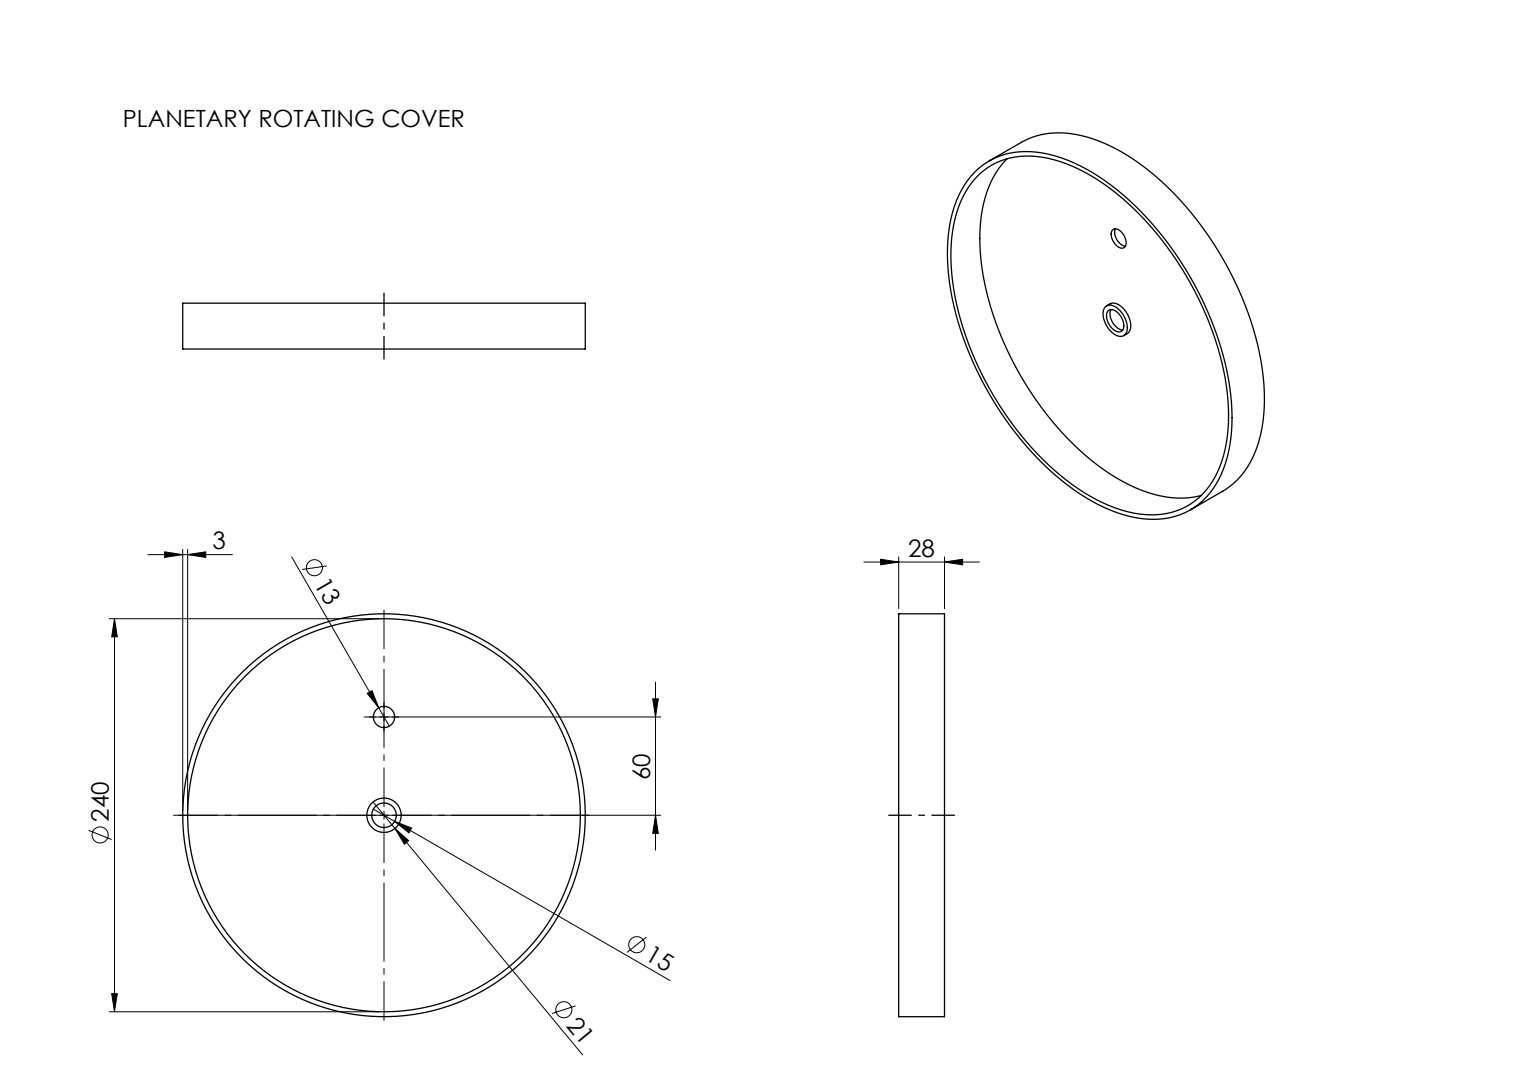
ISO-10303-21;
HEADER;
FILE_DESCRIPTION (('STEP AP214'),
    '1' );
FILE_NAME ('planetary rotating cover.step',
    '2026-09-30T13:58:28',
    ( '' ),
    ( '' ),
    'SwSTEP 2.0',
    'SolidWorks 2026',
    '' );
FILE_SCHEMA (( 'AUTOMOTIVE_DESIGN' ));
ENDSEC;

DATA;
#96=ORIENTED_EDGE ( 'NONE', *, *, #16353, .T. ) ;
#109=DIRECTION ( 'NONE',  ( -0.000000000000000000, -0.000000000000000000, 1.000000000000000000 ) ) ;
#161=ORIENTED_EDGE ( 'NONE', *, *, #12699, .T. ) ;
#178=ORIENTED_EDGE ( 'NONE', *, *, #6724, .F. ) ;
#209=EDGE_CURVE ( 'NONE', #16392, #6661, #15284, .T. ) ;
#268=CARTESIAN_POINT ( 'NONE',  ( 120.0000000000000000, 0.000000000000000000, -3.000000000000000000 ) ) ;
#330=CIRCLE ( 'NONE', #4199, 123.0000000000000000 ) ;
#469=CIRCLE ( 'NONE', #10677, 10.49999999999999822 ) ;
#487=CARTESIAN_POINT ( 'NONE',  ( 0.000000000000000000, 0.000000000000000000, 3.000000000000000000 ) ) ;
#587=FACE_OUTER_BOUND ( 'NONE', #12213, .T. ) ;
#707=DIRECTION ( 'NONE',  ( 0.000000000000000000, 0.000000000000000000, 1.000000000000000000 ) ) ;
#787=CARTESIAN_POINT ( 'NONE',  ( 0.000000000000000000, 0.000000000000000000, 25.00000000000000000 ) ) ;
#790=DIRECTION ( 'NONE',  ( -0.000000000000000000, -0.000000000000000000, -1.000000000000000000 ) ) ;
#853=ORIENTED_EDGE ( 'NONE', *, *, #4633, .T. ) ;
#891=FACE_OUTER_BOUND ( 'NONE', #4555, .T. ) ;
#949=FACE_OUTER_BOUND ( 'NONE', #6336, .T. ) ;
#1071=CARTESIAN_POINT ( 'NONE',  ( 6.499999999999984901, 60.00000000000001421, -3.000000000000000000 ) ) ;
#1097=EDGE_CURVE ( 'NONE', #6661, #9836, #21450, .T. ) ;
#1153=MECHANICAL_DESIGN_GEOMETRIC_PRESENTATION_REPRESENTATION('',(#14569),#20227);
#1202=DIRECTION ( 'NONE',  ( 0.000000000000000000, 0.000000000000000000, 1.000000000000000000 ) ) ;
#1264=CLOSED_SHELL ( 'NONE', ( #11800, #19951, #12732, #8634, #1598, #8913, #1358, #1778, #18719, #8874, #10287, #11609, #3169, #12589, #21642 ) ) ;
#1356=CYLINDRICAL_SURFACE ( 'NONE', #13917, 120.0000000000000000 ) ;
#1358=ADVANCED_FACE ( 'NONE', ( #13091 ), #3256, .T. ) ;
#1431=DIRECTION ( 'NONE',  ( 1.000000000000000000, 0.000000000000000000, 0.000000000000000000 ) ) ;
#1460=DIRECTION ( 'NONE',  ( 0.000000000000000000, 0.000000000000000000, 1.000000000000000000 ) ) ;
#1466=DIRECTION ( 'NONE',  ( 0.000000000000000000, 0.000000000000000000, 1.000000000000000000 ) ) ;
#1469=ORIENTED_EDGE ( 'NONE', *, *, #19172, .F. ) ;
#1491=EDGE_CURVE ( 'NONE', #2109, #20211, #15614, .T. ) ;
#1495=UNCERTAINTY_MEASURE_WITH_UNIT (LENGTH_MEASURE( 1.000000000000000082E-05 ), #15175, 'distance_accuracy_value', 'NONE');
#1560=AXIS2_PLACEMENT_3D ( 'NONE', #18307, #3156, #9890 ) ;
#1575=DIRECTION ( 'NONE',  ( -0.000000000000000000, -0.000000000000000000, 1.000000000000000000 ) ) ;
#1580=ORIENTED_EDGE ( 'NONE', *, *, #18346, .T. ) ;
#1598=ADVANCED_FACE ( 'NONE', ( #11080 ), #19377, .F. ) ;
#1657=CARTESIAN_POINT ( 'NONE',  ( -1.500346250137462226E-14, 60.00000000000001421, 0.000000000000000000 ) ) ;
#1704=ORIENTED_EDGE ( 'NONE', *, *, #7014, .F. ) ;
#1705=SURFACE_SIDE_STYLE ('',( #16621 ) ) ;
#1778=ADVANCED_FACE ( 'NONE', ( #6239, #21681 ), #14615, .F. ) ;
#1801=DIRECTION ( 'NONE',  ( -0.000000000000000000, -0.000000000000000000, -1.000000000000000000 ) ) ;
#1816=( GEOMETRIC_REPRESENTATION_CONTEXT ( 3 ) GLOBAL_UNCERTAINTY_ASSIGNED_CONTEXT ( ( #1495 ) ) GLOBAL_UNIT_ASSIGNED_CONTEXT ( ( #15175, #13183, #5240 ) ) REPRESENTATION_CONTEXT ( 'NONE', 'WORKASPACE' ) );
#1818=DIRECTION ( 'NONE',  ( 0.000000000000000000, 0.000000000000000000, 1.000000000000000000 ) ) ;
#1872=DIRECTION ( 'NONE',  ( -1.000000000000000000, 0.000000000000000000, 0.000000000000000000 ) ) ;
#1914=SHAPE_REPRESENTATION_RELATIONSHIP ( 'NONE' , 'NONE' ,  #4577, #5094 ) ;
#2060=VERTEX_POINT ( 'NONE', #2333 ) ;
#2094=EDGE_CURVE ( 'NONE', #19024, #4094, #17398, .T. ) ;
#2109=VERTEX_POINT ( 'NONE', #4756 ) ;
#2126=DIRECTION ( 'NONE',  ( 0.000000000000000000, 0.000000000000000000, 1.000000000000000000 ) ) ;
#2145=AXIS2_PLACEMENT_3D ( 'NONE', #2847, #9561, #14882 ) ;
#2162=EDGE_CURVE ( 'NONE', #4580, #18259, #11611, .T. ) ;
#2194=SURFACE_SIDE_STYLE ('',( #3536 ) ) ;
#2221=CARTESIAN_POINT ( 'NONE',  ( -1.500346250137462226E-14, 60.00000000000001421, 0.000000000000000000 ) ) ;
#2238=AXIS2_PLACEMENT_3D ( 'NONE', #19920, #1466, #14942 ) ;
#2256=EDGE_LOOP ( 'NONE', ( #9104, #1580, #6007, #10175 ) ) ;
#2333=CARTESIAN_POINT ( 'NONE',  ( 10.49999999999999822, 1.285879139104720633E-15, 3.000000000000000000 ) ) ;
#2468=CARTESIAN_POINT ( 'NONE',  ( 0.000000000000000000, 0.000000000000000000, 0.000000000000000000 ) ) ;
#2481=EDGE_LOOP ( 'NONE', ( #13688, #16346 ) ) ;
#2596=VERTEX_POINT ( 'NONE', #21507 ) ;
#2605=AXIS2_PLACEMENT_3D ( 'NONE', #6887, #1575, #5000 ) ;
#2665=AXIS2_PLACEMENT_3D ( 'NONE', #11325, #16849, #3369 ) ;
#2847=CARTESIAN_POINT ( 'NONE',  ( 0.000000000000000000, 0.000000000000000000, 0.000000000000000000 ) ) ;
#2895=PRODUCT_CONTEXT ( 'NONE', #11362, 'mechanical' ) ;
#2899=DIRECTION ( 'NONE',  ( 0.000000000000000000, 0.000000000000000000, 1.000000000000000000 ) ) ;
#2977=VERTEX_POINT ( 'NONE', #16386 ) ;
#2997=EDGE_LOOP ( 'NONE', ( #5307, #12866, #1469, #19939 ) ) ;
#2999=CIRCLE ( 'NONE', #5835, 6.500000000000000000 ) ;
#3008=CARTESIAN_POINT ( 'NONE',  ( 123.0000000000000000, 0.000000000000000000, 25.00000000000000000 ) ) ;
#3051=UNCERTAINTY_MEASURE_WITH_UNIT (LENGTH_MEASURE( 1.000000000000000082E-05 ), #12039, 'distance_accuracy_value', 'NONE');
#3156=DIRECTION ( 'NONE',  ( 0.000000000000000000, 0.000000000000000000, 1.000000000000000000 ) ) ;
#3169=ADVANCED_FACE ( 'NONE', ( #10296 ), #18600, .T. ) ;
#3229=( GEOMETRIC_REPRESENTATION_CONTEXT ( 3 ) GLOBAL_UNCERTAINTY_ASSIGNED_CONTEXT ( ( #18310 ) ) GLOBAL_UNIT_ASSIGNED_CONTEXT ( ( #3244, #5015, #3469 ) ) REPRESENTATION_CONTEXT ( 'NONE', 'WORKASPACE' ) );
#3244=( LENGTH_UNIT ( ) NAMED_UNIT ( * ) SI_UNIT ( .MILLI., .METRE. ) );
#3256=CYLINDRICAL_SURFACE ( 'NONE', #17531, 123.0000000000000000 ) ;
#3298=CARTESIAN_POINT ( 'NONE',  ( 0.000000000000000000, 0.000000000000000000, 0.000000000000000000 ) ) ;
#3309=DIRECTION ( 'NONE',  ( -1.000000000000000000, 0.000000000000000000, 0.000000000000000000 ) ) ;
#3339=CARTESIAN_POINT ( 'NONE',  ( 0.000000000000000000, 0.000000000000000000, 3.000000000000000000 ) ) ;
#3369=DIRECTION ( 'NONE',  ( -1.000000000000000000, 0.000000000000000000, 0.000000000000000000 ) ) ;
#3469=( NAMED_UNIT ( * ) SI_UNIT ( $, .STERADIAN. ) SOLID_ANGLE_UNIT ( ) );
#3536=SURFACE_STYLE_FILL_AREA ( #18684 ) ;
#3553=VERTEX_POINT ( 'NONE', #15468 ) ;
#3586=CARTESIAN_POINT ( 'NONE',  ( -10.49999999999999822, 0.000000000000000000, 3.000000000000000000 ) ) ;
#3631=ORIENTED_EDGE ( 'NONE', *, *, #16907, .F. ) ;
#3797=DIRECTION ( 'NONE',  ( 0.000000000000000000, 0.000000000000000000, -1.000000000000000000 ) ) ;
#3837=CIRCLE ( 'NONE', #11249, 6.500000000000000000 ) ;
#3899=ORIENTED_EDGE ( 'NONE', *, *, #8911, .T. ) ;
#3934=DIRECTION ( 'NONE',  ( 1.000000000000000000, 0.000000000000000000, 0.000000000000000000 ) ) ;
#3999=PLANE ( 'NONE',  #7015 ) ;
#4005=ORIENTED_EDGE ( 'NONE', *, *, #2162, .F. ) ;
#4042=CARTESIAN_POINT ( 'NONE',  ( 0.000000000000000000, 0.000000000000000000, 3.000000000000000000 ) ) ;
#4065=ORIENTED_EDGE ( 'NONE', *, *, #11624, .F. ) ;
#4094=VERTEX_POINT ( 'NONE', #3008 ) ;
#4199=AXIS2_PLACEMENT_3D ( 'NONE', #4946, #21614, #21520 ) ;
#4212=DIRECTION ( 'NONE',  ( -1.000000000000000000, 0.000000000000000000, 0.000000000000000000 ) ) ;
#4216=VECTOR ( 'NONE', #20851, 1000.000000000000000 ) ;
#4340=DIRECTION ( 'NONE',  ( 1.000000000000000000, 0.000000000000000000, 0.000000000000000000 ) ) ;
#4401=( NAMED_UNIT ( * ) SI_UNIT ( $, .STERADIAN. ) SOLID_ANGLE_UNIT ( ) );
#4555=EDGE_LOOP ( 'NONE', ( #10212, #7117, #8225, #4005 ) ) ;
#4577=SHAPE_REPRESENTATION ( 'planetary rotating cover', ( #15567 ), #3229 ) ;
#4580=VERTEX_POINT ( 'NONE', #6752 ) ;
#4597=FACE_OUTER_BOUND ( 'NONE', #12724, .T. ) ;
#4633=EDGE_CURVE ( 'NONE', #20616, #7569, #3837, .T. ) ;
#4756=CARTESIAN_POINT ( 'NONE',  ( -10.49999999999999822, 0.000000000000000000, 3.000000000000000000 ) ) ;
#4797=CARTESIAN_POINT ( 'NONE',  ( -120.0000000000000000, 1.469576158976823671E-14, -3.000000000000000000 ) ) ;
#4899=VECTOR ( 'NONE', #16580, 1000.000000000000000 ) ;
#4936=VECTOR ( 'NONE', #19718, 1000.000000000000000 ) ;
#4946=CARTESIAN_POINT ( 'NONE',  ( 0.000000000000000000, 0.000000000000000000, 25.00000000000000000 ) ) ;
#4999=COLOUR_RGB ( '', 0.66274510, 0.83137255, 0.94901961) ;
#5000=DIRECTION ( 'NONE',  ( -1.000000000000000000, 0.000000000000000000, 0.000000000000000000 ) ) ;
#5015=( NAMED_UNIT ( * ) PLANE_ANGLE_UNIT ( ) SI_UNIT ( $, .RADIAN. ) );
#5028=LINE ( 'NONE', #8346, #11852 ) ;
#5090=CARTESIAN_POINT ( 'NONE',  ( 0.000000000000000000, 0.000000000000000000, -3.000000000000000000 ) ) ;
#5094=ADVANCED_BREP_SHAPE_REPRESENTATION ( '', ( #6054, #15567 ), #3229 ) ;
#5199=ORIENTED_EDGE ( 'NONE', *, *, #2094, .F. ) ;
#5240=( NAMED_UNIT ( * ) SI_UNIT ( $, .STERADIAN. ) SOLID_ANGLE_UNIT ( ) );
#5269=EDGE_CURVE ( 'NONE', #4580, #12701, #7733, .T. ) ;
#5298=DIRECTION ( 'NONE',  ( 0.000000000000000000, 0.000000000000000000, 1.000000000000000000 ) ) ;
#5307=ORIENTED_EDGE ( 'NONE', *, *, #14907, .T. ) ;
#5462=FACE_BOUND ( 'NONE', #10495, .T. ) ;
#5468=AXIS2_PLACEMENT_3D ( 'NONE', #3298, #1202, #1431 ) ;
#5486=ORIENTED_EDGE ( 'NONE', *, *, #13236, .F. ) ;
#5501=CARTESIAN_POINT ( 'NONE',  ( 7.500000000000000000, 9.184850993605147944E-16, 3.000000000000000000 ) ) ;
#5548=CYLINDRICAL_SURFACE ( 'NONE', #15020, 7.500000000000000000 ) ;
#5565=ORIENTED_EDGE ( 'NONE', *, *, #10122, .T. ) ;
#5568=DIRECTION ( 'NONE',  ( 0.000000000000000000, 0.000000000000000000, 1.000000000000000000 ) ) ;
#5737=FILL_AREA_STYLE_COLOUR ( '', #9601 ) ;
#5835=AXIS2_PLACEMENT_3D ( 'NONE', #2221, #8747, #4212 ) ;
#6005=FACE_BOUND ( 'NONE', #2481, .T. ) ;
#6007=ORIENTED_EDGE ( 'NONE', *, *, #10276, .T. ) ;
#6012=ORIENTED_EDGE ( 'NONE', *, *, #10919, .T. ) ;
#6054=MANIFOLD_SOLID_BREP ( 'Extrude-Thin2', #1264 ) ;
#6110=CARTESIAN_POINT ( 'NONE',  ( 0.000000000000000000, 0.000000000000000000, 3.000000000000000000 ) ) ;
#6117=CARTESIAN_POINT ( 'NONE',  ( -1.500346250137462226E-14, 60.00000000000001421, -3.000000000000000000 ) ) ;
#6181=AXIS2_PLACEMENT_3D ( 'NONE', #12406, #10750, #9100 ) ;
#6239=FACE_OUTER_BOUND ( 'NONE', #9790, .T. ) ;
#6268=DIRECTION ( 'NONE',  ( 0.000000000000000000, 0.000000000000000000, -1.000000000000000000 ) ) ;
#6336=EDGE_LOOP ( 'NONE', ( #21615, #5565, #15308, #9420 ) ) ;
#6419=EDGE_LOOP ( 'NONE', ( #14085, #6523 ) ) ;
#6445=EDGE_LOOP ( 'NONE', ( #10849, #21171 ) ) ;
#6523=ORIENTED_EDGE ( 'NONE', *, *, #10122, .F. ) ;
#6573=DIRECTION ( 'NONE',  ( -0.000000000000000000, -0.000000000000000000, 1.000000000000000000 ) ) ;
#6661=VERTEX_POINT ( 'NONE', #21601 ) ;
#6710=DIRECTION ( 'NONE',  ( 1.000000000000000000, 0.000000000000000000, 0.000000000000000000 ) ) ;
#6724=EDGE_CURVE ( 'NONE', #2060, #2109, #14249, .T. ) ;
#6752=CARTESIAN_POINT ( 'NONE',  ( -7.500000000000000000, 0.000000000000000000, 3.000000000000000000 ) ) ;
#6826=AXIS2_PLACEMENT_3D ( 'NONE', #7636, #14373, #18029 ) ;
#6848=EDGE_LOOP ( 'NONE', ( #96, #12052 ) ) ;
#6887=CARTESIAN_POINT ( 'NONE',  ( 0.000000000000000000, 0.000000000000000000, 0.000000000000000000 ) ) ;
#6896=AXIS2_PLACEMENT_3D ( 'NONE', #18158, #1460, #4340 ) ;
#6909=LINE ( 'NONE', #21702, #16378 ) ;
#7014=EDGE_CURVE ( 'NONE', #8843, #3553, #13566, .T. ) ;
#7015=AXIS2_PLACEMENT_3D ( 'NONE', #787, #14264, #21017 ) ;
#7017=CYLINDRICAL_SURFACE ( 'NONE', #12838, 123.0000000000000000 ) ;
#7117=ORIENTED_EDGE ( 'NONE', *, *, #15442, .T. ) ;
#7181=DIRECTION ( 'NONE',  ( 1.000000000000000000, 0.000000000000000000, 0.000000000000000000 ) ) ;
#7238=AXIS2_PLACEMENT_3D ( 'NONE', #487, #12199, #13965 ) ;
#7281=APPLICATION_CONTEXT ( 'automotive_design' ) ;
#7286=CIRCLE ( 'NONE', #21397, 6.500000000000000000 ) ;
#7556=ORIENTED_EDGE ( 'NONE', *, *, #13083, .F. ) ;
#7569=VERTEX_POINT ( 'NONE', #11910 ) ;
#7595=AXIS2_PLACEMENT_3D ( 'NONE', #7995, #19917, #14725 ) ;
#7636=CARTESIAN_POINT ( 'NONE',  ( 0.000000000000000000, 0.000000000000000000, 25.00000000000000000 ) ) ;
#7640=DIRECTION ( 'NONE',  ( -0.000000000000000000, -0.000000000000000000, -1.000000000000000000 ) ) ;
#7652=DIRECTION ( 'NONE',  ( -1.000000000000000000, 0.000000000000000000, 0.000000000000000000 ) ) ;
#7691=DIRECTION ( 'NONE',  ( -0.000000000000000000, -0.000000000000000000, -1.000000000000000000 ) ) ;
#7733=CIRCLE ( 'NONE', #16201, 7.500000000000000000 ) ;
#7834=ORIENTED_EDGE ( 'NONE', *, *, #4633, .F. ) ;
#7882=DIRECTION ( 'NONE',  ( 1.000000000000000000, 0.000000000000000000, -0.000000000000000000 ) ) ;
#7926=CIRCLE ( 'NONE', #7238, 7.500000000000000000 ) ;
#7995=CARTESIAN_POINT ( 'NONE',  ( -1.500346250137462226E-14, 60.00000000000001421, 0.000000000000000000 ) ) ;
#8066=EDGE_LOOP ( 'NONE', ( #19417, #4065, #16313, #19579 ) ) ;
#8225=ORIENTED_EDGE ( 'NONE', *, *, #16353, .F. ) ;
#8251=VERTEX_POINT ( 'NONE', #12007 ) ;
#8345=DIRECTION ( 'NONE',  ( 0.000000000000000000, 0.000000000000000000, 1.000000000000000000 ) ) ;
#8346=CARTESIAN_POINT ( 'NONE',  ( 6.499999999999984901, 60.00000000000001421, 0.000000000000000000 ) ) ;
#8406=EDGE_CURVE ( 'NONE', #8251, #16392, #20607, .T. ) ;
#8601=ORIENTED_EDGE ( 'NONE', *, *, #7014, .T. ) ;
#8634=ADVANCED_FACE ( 'NONE', ( #11981 ), #7017, .T. ) ;
#8685=EDGE_CURVE ( 'NONE', #8843, #19024, #6909, .T. ) ;
#8727=PRODUCT_DEFINITION_CONTEXT ( 'detailed design', #7281, 'design' ) ;
#8747=DIRECTION ( 'NONE',  ( 0.000000000000000000, 0.000000000000000000, -1.000000000000000000 ) ) ;
#8770=CARTESIAN_POINT ( 'NONE',  ( -123.0000000000000000, 1.506315562951244531E-14, -3.000000000000000000 ) ) ;
#8843=VERTEX_POINT ( 'NONE', #8770 ) ;
#8874=ADVANCED_FACE ( 'NONE', ( #10636, #5462, #17386 ), #13848, .F. ) ;
#8911=EDGE_CURVE ( 'NONE', #17874, #2596, #11811, .T. ) ;
#8913=ADVANCED_FACE ( 'NONE', ( #16162 ), #1356, .F. ) ;
#8966=FACE_OUTER_BOUND ( 'NONE', #6445, .T. ) ;
#8992=EDGE_LOOP ( 'NONE', ( #11317, #12388 ) ) ;
#9003=DIRECTION ( 'NONE',  ( -1.000000000000000000, 0.000000000000000000, 0.000000000000000000 ) ) ;
#9100=DIRECTION ( 'NONE',  ( 1.000000000000000000, 0.000000000000000000, 0.000000000000000000 ) ) ;
#9104=ORIENTED_EDGE ( 'NONE', *, *, #8406, .F. ) ;
#9193=DIRECTION ( 'NONE',  ( -1.000000000000000000, 0.000000000000000000, -0.000000000000000000 ) ) ;
#9332=CARTESIAN_POINT ( 'NONE',  ( 0.000000000000000000, 0.000000000000000000, 25.00000000000000000 ) ) ;
#9345=CARTESIAN_POINT ( 'NONE',  ( -6.500000000000014211, 60.00000000000001421, 0.000000000000000000 ) ) ;
#9409=CARTESIAN_POINT ( 'NONE',  ( -1.500346250137462226E-14, 60.00000000000001421, -3.000000000000000000 ) ) ;
#9420=ORIENTED_EDGE ( 'NONE', *, *, #9740, .F. ) ;
#9522=CARTESIAN_POINT ( 'NONE',  ( 0.000000000000000000, 0.000000000000000000, 3.000000000000000000 ) ) ;
#9561=DIRECTION ( 'NONE',  ( 0.000000000000000000, 0.000000000000000000, -1.000000000000000000 ) ) ;
#9601=COLOUR_RGB ( '', 0.66274510, 0.83137255, 0.94901961) ;
#9615=SHAPE_DEFINITION_REPRESENTATION ( #17096, #4577 ) ;
#9738=DIRECTION ( 'NONE',  ( 0.000000000000000000, 0.000000000000000000, 1.000000000000000000 ) ) ;
#9740=EDGE_CURVE ( 'NONE', #15128, #18259, #21674, .T. ) ;
#9741=FACE_OUTER_BOUND ( 'NONE', #20137, .T. ) ;
#9789=FACE_OUTER_BOUND ( 'NONE', #6848, .T. ) ;
#9790=EDGE_LOOP ( 'NONE', ( #10417, #1704 ) ) ;
#9836=VERTEX_POINT ( 'NONE', #16195 ) ;
#9890=DIRECTION ( 'NONE',  ( 1.000000000000000000, 0.000000000000000000, 0.000000000000000000 ) ) ;
#9986=CARTESIAN_POINT ( 'NONE',  ( 0.000000000000000000, 0.000000000000000000, -3.000000000000000000 ) ) ;
#10063=ORIENTED_EDGE ( 'NONE', *, *, #16907, .T. ) ;
#10111=LINE ( 'NONE', #19248, #19257 ) ;
#10122=EDGE_CURVE ( 'NONE', #12701, #4580, #7926, .T. ) ;
#10155=AXIS2_PLACEMENT_3D ( 'NONE', #11191, #707, #17509 ) ;
#10175=ORIENTED_EDGE ( 'NONE', *, *, #209, .F. ) ;
#10196=CARTESIAN_POINT ( 'NONE',  ( 0.000000000000000000, 0.000000000000000000, 3.000000000000000000 ) ) ;
#10209=SURFACE_STYLE_USAGE ( .BOTH. , #1705 ) ;
#10212=ORIENTED_EDGE ( 'NONE', *, *, #5269, .T. ) ;
#10276=EDGE_CURVE ( 'NONE', #9836, #6661, #16057, .T. ) ;
#10287=ADVANCED_FACE ( 'NONE', ( #9741 ), #16381, .F. ) ;
#10296=FACE_OUTER_BOUND ( 'NONE', #18535, .T. ) ;
#10311=DIRECTION ( 'NONE',  ( 0.000000000000000000, 0.000000000000000000, 1.000000000000000000 ) ) ;
#10359=CIRCLE ( 'NONE', #2605, 120.0000000000000000 ) ;
#10369=( NAMED_UNIT ( * ) PLANE_ANGLE_UNIT ( ) SI_UNIT ( $, .RADIAN. ) );
#10376=DIRECTION ( 'NONE',  ( 0.000000000000000000, 0.000000000000000000, 1.000000000000000000 ) ) ;
#10417=ORIENTED_EDGE ( 'NONE', *, *, #14907, .F. ) ;
#10495=EDGE_LOOP ( 'NONE', ( #853, #15182 ) ) ;
#10575=EDGE_CURVE ( 'NONE', #7569, #20616, #2999, .T. ) ;
#10635=MECHANICAL_DESIGN_GEOMETRIC_PRESENTATION_REPRESENTATION('',(#17355),#1816);
#10636=FACE_BOUND ( 'NONE', #18431, .T. ) ;
#10663=DIRECTION ( 'NONE',  ( -0.000000000000000000, -0.000000000000000000, 1.000000000000000000 ) ) ;
#10677=AXIS2_PLACEMENT_3D ( 'NONE', #17014, #109, #1872 ) ;
#10711=ORIENTED_EDGE ( 'NONE', *, *, #10575, .F. ) ;
#10750=DIRECTION ( 'NONE',  ( 0.000000000000000000, 0.000000000000000000, 1.000000000000000000 ) ) ;
#10845=VECTOR ( 'NONE', #16614, 1000.000000000000000 ) ;
#10849=ORIENTED_EDGE ( 'NONE', *, *, #19172, .T. ) ;
#10919=EDGE_CURVE ( 'NONE', #2977, #20211, #469, .T. ) ;
#11075=DIRECTION ( 'NONE',  ( -1.000000000000000000, 0.000000000000000000, 0.000000000000000000 ) ) ;
#11080=FACE_OUTER_BOUND ( 'NONE', #2256, .T. ) ;
#11191=CARTESIAN_POINT ( 'NONE',  ( 0.000000000000000000, 0.000000000000000000, -3.000000000000000000 ) ) ;
#11249=AXIS2_PLACEMENT_3D ( 'NONE', #1657, #15021, #3309 ) ;
#11317=ORIENTED_EDGE ( 'NONE', *, *, #11624, .T. ) ;
#11325=CARTESIAN_POINT ( 'NONE',  ( -1.500346250137462226E-14, 60.00000000000001421, 0.000000000000000000 ) ) ;
#11362=APPLICATION_CONTEXT ( 'automotive_design' ) ;
#11423=PRODUCT ( 'planetary rotating cover', 'planetary rotating cover', '', ( #2895 ) ) ;
#11609=ADVANCED_FACE ( 'NONE', ( #13170, #12844 ), #16605, .T. ) ;
#11611=LINE ( 'NONE', #18131, #4899 ) ;
#11613=EDGE_CURVE ( 'NONE', #20211, #2977, #18845, .T. ) ;
#11619=AXIS2_PLACEMENT_3D ( 'NONE', #5090, #10376, #7181 ) ;
#11624=EDGE_CURVE ( 'NONE', #16392, #8251, #10359, .T. ) ;
#11629=ORIENTED_EDGE ( 'NONE', *, *, #13083, .T. ) ;
#11640=CARTESIAN_POINT ( 'NONE',  ( 0.000000000000000000, 0.000000000000000000, -3.000000000000000000 ) ) ;
#11800=ADVANCED_FACE ( 'NONE', ( #891 ), #5548, .F. ) ;
#11811=CIRCLE ( 'NONE', #16022, 6.500000000000000000 ) ;
#11852=VECTOR ( 'NONE', #6268, 1000.000000000000000 ) ;
#11860=ORIENTED_EDGE ( 'NONE', *, *, #8685, .F. ) ;
#11870=DIRECTION ( 'NONE',  ( 1.000000000000000000, 0.000000000000000000, 0.000000000000000000 ) ) ;
#11910=CARTESIAN_POINT ( 'NONE',  ( 6.499999999999984901, 60.00000000000001421, 0.000000000000000000 ) ) ;
#11929=VECTOR ( 'NONE', #18837, 1000.000000000000000 ) ;
#11981=FACE_OUTER_BOUND ( 'NONE', #2997, .T. ) ;
#12007=CARTESIAN_POINT ( 'NONE',  ( -120.0000000000000000, 1.469576158976823671E-14, 0.000000000000000000 ) ) ;
#12027=LINE ( 'NONE', #20106, #15475 ) ;
#12039=( LENGTH_UNIT ( ) NAMED_UNIT ( * ) SI_UNIT ( .MILLI., .METRE. ) );
#12052=ORIENTED_EDGE ( 'NONE', *, *, #9740, .T. ) ;
#12131=AXIS2_PLACEMENT_3D ( 'NONE', #21683, #6573, #20147 ) ;
#12199=DIRECTION ( 'NONE',  ( 0.000000000000000000, 0.000000000000000000, 1.000000000000000000 ) ) ;
#12213=EDGE_LOOP ( 'NONE', ( #178, #16189, #6012, #15536 ) ) ;
#12305=CIRCLE ( 'NONE', #11619, 123.0000000000000000 ) ;
#12385=DIRECTION ( 'NONE',  ( -1.000000000000000000, 0.000000000000000000, 0.000000000000000000 ) ) ;
#12388=ORIENTED_EDGE ( 'NONE', *, *, #8406, .T. ) ;
#12406=CARTESIAN_POINT ( 'NONE',  ( 0.000000000000000000, 0.000000000000000000, -3.000000000000000000 ) ) ;
#12589=ADVANCED_FACE ( 'NONE', ( #949 ), #12874, .F. ) ;
#12699=EDGE_CURVE ( 'NONE', #7569, #17874, #5028, .T. ) ;
#12701=VERTEX_POINT ( 'NONE', #12986 ) ;
#12724=EDGE_LOOP ( 'NONE', ( #10711, #161, #3899, #3631 ) ) ;
#12732=ADVANCED_FACE ( 'NONE', ( #4597 ), #18190, .F. ) ;
#12758=CARTESIAN_POINT ( 'NONE',  ( 0.000000000000000000, 0.000000000000000000, 0.000000000000000000 ) ) ;
#12768=VECTOR ( 'NONE', #5568, 1000.000000000000000 ) ;
#12838=AXIS2_PLACEMENT_3D ( 'NONE', #20273, #1818, #11870 ) ;
#12844=FACE_BOUND ( 'NONE', #6419, .T. ) ;
#12866=ORIENTED_EDGE ( 'NONE', *, *, #8685, .T. ) ;
#12873=DIRECTION ( 'NONE',  ( 1.000000000000000000, 0.000000000000000000, 0.000000000000000000 ) ) ;
#12874=CYLINDRICAL_SURFACE ( 'NONE', #15003, 7.500000000000000000 ) ;
#12986=CARTESIAN_POINT ( 'NONE',  ( 7.500000000000000000, 9.184850993605147944E-16, 3.000000000000000000 ) ) ;
#13063=DIRECTION ( 'NONE',  ( 1.000000000000000000, 0.000000000000000000, 0.000000000000000000 ) ) ;
#13083=EDGE_CURVE ( 'NONE', #2596, #17874, #7286, .T. ) ;
#13091=FACE_OUTER_BOUND ( 'NONE', #15281, .T. ) ;
#13170=FACE_OUTER_BOUND ( 'NONE', #20579, .T. ) ;
#13180=CARTESIAN_POINT ( 'NONE',  ( 10.49999999999999822, 1.285879139104720633E-15, 3.000000000000000000 ) ) ;
#13183=( NAMED_UNIT ( * ) PLANE_ANGLE_UNIT ( ) SI_UNIT ( $, .RADIAN. ) );
#13207=ORIENTED_EDGE ( 'NONE', *, *, #11613, .F. ) ;
#13236=EDGE_CURVE ( 'NONE', #2109, #2060, #17519, .T. ) ;
#13358=EDGE_LOOP ( 'NONE', ( #7556, #19618 ) ) ;
#13483=CARTESIAN_POINT ( 'NONE',  ( -10.49999999999999822, 0.000000000000000000, 0.000000000000000000 ) ) ;
#13566=CIRCLE ( 'NONE', #6181, 123.0000000000000000 ) ;
#13596=AXIS2_PLACEMENT_3D ( 'NONE', #6110, #790, #7652 ) ;
#13688=ORIENTED_EDGE ( 'NONE', *, *, #1097, .F. ) ;
#13790=CARTESIAN_POINT ( 'NONE',  ( 120.0000000000000000, 0.000000000000000000, 0.000000000000000000 ) ) ;
#13848=PLANE ( 'NONE',  #19915 ) ;
#13917=AXIS2_PLACEMENT_3D ( 'NONE', #21247, #2899, #17825 ) ;
#13965=DIRECTION ( 'NONE',  ( 1.000000000000000000, 0.000000000000000000, 0.000000000000000000 ) ) ;
#14085=ORIENTED_EDGE ( 'NONE', *, *, #5269, .F. ) ;
#14249=CIRCLE ( 'NONE', #1560, 10.49999999999999822 ) ;
#14264=DIRECTION ( 'NONE',  ( 0.000000000000000000, 0.000000000000000000, 1.000000000000000000 ) ) ;
#14282=DIRECTION ( 'NONE',  ( -1.000000000000000000, 0.000000000000000000, 0.000000000000000000 ) ) ;
#14373=DIRECTION ( 'NONE',  ( 0.000000000000000000, 0.000000000000000000, 1.000000000000000000 ) ) ;
#14569=STYLED_ITEM ( 'NONE', ( #15672 ), #6054 ) ;
#14615=PLANE ( 'NONE',  #20238 ) ;
#14725=DIRECTION ( 'NONE',  ( -1.000000000000000000, 0.000000000000000000, 0.000000000000000000 ) ) ;
#14803=ORIENTED_EDGE ( 'NONE', *, *, #1491, .T. ) ;
#14831=DIRECTION ( 'NONE',  ( 0.000000000000000000, 0.000000000000000000, -1.000000000000000000 ) ) ;
#14882=DIRECTION ( 'NONE',  ( -1.000000000000000000, 0.000000000000000000, -0.000000000000000000 ) ) ;
#14907=EDGE_CURVE ( 'NONE', #3553, #8843, #12305, .T. ) ;
#14942=DIRECTION ( 'NONE',  ( 1.000000000000000000, 0.000000000000000000, -0.000000000000000000 ) ) ;
#14970=AXIS2_PLACEMENT_3D ( 'NONE', #12758, #17748, #3934 ) ;
#15003=AXIS2_PLACEMENT_3D ( 'NONE', #4042, #7691, #20844 ) ;
#15020=AXIS2_PLACEMENT_3D ( 'NONE', #19241, #7640, #12385 ) ;
#15021=DIRECTION ( 'NONE',  ( 0.000000000000000000, 0.000000000000000000, -1.000000000000000000 ) ) ;
#15128=VERTEX_POINT ( 'NONE', #20872 ) ;
#15175=( LENGTH_UNIT ( ) NAMED_UNIT ( * ) SI_UNIT ( .MILLI., .METRE. ) );
#15182=ORIENTED_EDGE ( 'NONE', *, *, #10575, .T. ) ;
#15281=EDGE_LOOP ( 'NONE', ( #11860, #8601, #20023, #5199 ) ) ;
#15284=LINE ( 'NONE', #268, #12768 ) ;
#15308=ORIENTED_EDGE ( 'NONE', *, *, #2162, .T. ) ;
#15342=SURFACE_STYLE_USAGE ( .BOTH. , #2194 ) ;
#15442=EDGE_CURVE ( 'NONE', #12701, #15128, #17326, .T. ) ;
#15461=AXIS2_PLACEMENT_3D ( 'NONE', #9332, #17645, #12873 ) ;
#15468=CARTESIAN_POINT ( 'NONE',  ( 123.0000000000000000, 0.000000000000000000, -3.000000000000000000 ) ) ;
#15475=VECTOR ( 'NONE', #5298, 1000.000000000000000 ) ;
#15536=ORIENTED_EDGE ( 'NONE', *, *, #1491, .F. ) ;
#15567=AXIS2_PLACEMENT_3D ( 'NONE', #21837, #20187, #17085 ) ;
#15614=LINE ( 'NONE', #3586, #11929 ) ;
#15672=PRESENTATION_STYLE_ASSIGNMENT (( #15342 ) ) ;
#15743=AXIS2_PLACEMENT_3D ( 'NONE', #3339, #2126, #17268 ) ;
#16022=AXIS2_PLACEMENT_3D ( 'NONE', #6117, #14831, #11075 ) ;
#16057=CIRCLE ( 'NONE', #6896, 120.0000000000000000 ) ;
#16154=CYLINDRICAL_SURFACE ( 'NONE', #13596, 10.49999999999999822 ) ;
#16162=FACE_OUTER_BOUND ( 'NONE', #8066, .T. ) ;
#16189=ORIENTED_EDGE ( 'NONE', *, *, #19619, .T. ) ;
#16195=CARTESIAN_POINT ( 'NONE',  ( -120.0000000000000000, 1.469576158976823671E-14, 25.00000000000000000 ) ) ;
#16201=AXIS2_PLACEMENT_3D ( 'NONE', #9522, #9738, #13063 ) ;
#16265=ORIENTED_EDGE ( 'NONE', *, *, #19619, .F. ) ;
#16313=ORIENTED_EDGE ( 'NONE', *, *, #209, .T. ) ;
#16346=ORIENTED_EDGE ( 'NONE', *, *, #10276, .F. ) ;
#16353=EDGE_CURVE ( 'NONE', #18259, #15128, #20295, .T. ) ;
#16378=VECTOR ( 'NONE', #10311, 1000.000000000000000 ) ;
#16381=CYLINDRICAL_SURFACE ( 'NONE', #7595, 6.500000000000000000 ) ;
#16386=CARTESIAN_POINT ( 'NONE',  ( 10.49999999999999822, 1.285879139104720633E-15, 0.000000000000000000 ) ) ;
#16392=VERTEX_POINT ( 'NONE', #13790 ) ;
#16580=DIRECTION ( 'NONE',  ( -0.000000000000000000, -0.000000000000000000, -1.000000000000000000 ) ) ;
#16590=ORIENTED_EDGE ( 'NONE', *, *, #6724, .T. ) ;
#16605=PLANE ( 'NONE',  #2238 ) ;
#16614=DIRECTION ( 'NONE',  ( 0.000000000000000000, 0.000000000000000000, 1.000000000000000000 ) ) ;
#16621=SURFACE_STYLE_FILL_AREA ( #16837 ) ;
#16705=DIRECTION ( 'NONE',  ( 0.000000000000000000, 0.000000000000000000, 1.000000000000000000 ) ) ;
#16837=FILL_AREA_STYLE ('',( #17056 ) ) ;
#16849=DIRECTION ( 'NONE',  ( 0.000000000000000000, 0.000000000000000000, -1.000000000000000000 ) ) ;
#16856=DIRECTION ( 'NONE',  ( 0.000000000000000000, 0.000000000000000000, -1.000000000000000000 ) ) ;
#16907=EDGE_CURVE ( 'NONE', #20616, #2596, #10111, .T. ) ;
#16955=PRESENTATION_STYLE_ASSIGNMENT (( #10209 ) ) ;
#17014=CARTESIAN_POINT ( 'NONE',  ( 0.000000000000000000, 0.000000000000000000, 0.000000000000000000 ) ) ;
#17043=DIRECTION ( 'NONE',  ( -1.000000000000000000, 0.000000000000000000, 0.000000000000000000 ) ) ;
#17056=FILL_AREA_STYLE_COLOUR ( '', #4999 ) ;
#17078=AXIS2_PLACEMENT_3D ( 'NONE', #19076, #10663, #9003 ) ;
#17085=DIRECTION ( 'NONE',  ( 1.000000000000000000, 0.000000000000000000, 0.000000000000000000 ) ) ;
#17096=PRODUCT_DEFINITION_SHAPE ( 'NONE', 'NONE',  #19678 ) ;
#17268=DIRECTION ( 'NONE',  ( 1.000000000000000000, 0.000000000000000000, 0.000000000000000000 ) ) ;
#17326=LINE ( 'NONE', #5501, #4216 ) ;
#17355=STYLED_ITEM ( 'NONE', ( #16955 ), #5094 ) ;
#17386=FACE_OUTER_BOUND ( 'NONE', #8992, .T. ) ;
#17398=CIRCLE ( 'NONE', #6826, 123.0000000000000000 ) ;
#17438=CARTESIAN_POINT ( 'NONE',  ( -123.0000000000000000, 1.506315562951244531E-14, 25.00000000000000000 ) ) ;
#17509=DIRECTION ( 'NONE',  ( 1.000000000000000000, 0.000000000000000000, 0.000000000000000000 ) ) ;
#17519=CIRCLE ( 'NONE', #15743, 10.49999999999999822 ) ;
#17531=AXIS2_PLACEMENT_3D ( 'NONE', #9986, #8345, #6710 ) ;
#17645=DIRECTION ( 'NONE',  ( 0.000000000000000000, 0.000000000000000000, 1.000000000000000000 ) ) ;
#17697=PRODUCT_DEFINITION_FORMATION_WITH_SPECIFIED_SOURCE ( 'ANY', '', #11423, .NOT_KNOWN. ) ;
#17748=DIRECTION ( 'NONE',  ( 0.000000000000000000, 0.000000000000000000, 1.000000000000000000 ) ) ;
#17825=DIRECTION ( 'NONE',  ( 1.000000000000000000, 0.000000000000000000, 0.000000000000000000 ) ) ;
#17874=VERTEX_POINT ( 'NONE', #1071 ) ;
#17993=PLANE ( 'NONE',  #2145 ) ;
#18029=DIRECTION ( 'NONE',  ( 1.000000000000000000, 0.000000000000000000, 0.000000000000000000 ) ) ;
#18131=CARTESIAN_POINT ( 'NONE',  ( -7.500000000000000000, 0.000000000000000000, 3.000000000000000000 ) ) ;
#18158=CARTESIAN_POINT ( 'NONE',  ( 0.000000000000000000, 0.000000000000000000, 25.00000000000000000 ) ) ;
#18190=CYLINDRICAL_SURFACE ( 'NONE', #2665, 6.500000000000000000 ) ;
#18259=VERTEX_POINT ( 'NONE', #19390 ) ;
#18307=CARTESIAN_POINT ( 'NONE',  ( 0.000000000000000000, 0.000000000000000000, 3.000000000000000000 ) ) ;
#18310=UNCERTAINTY_MEASURE_WITH_UNIT (LENGTH_MEASURE( 1.000000000000000082E-05 ), #3244, 'distance_accuracy_value', 'NONE');
#18346=EDGE_CURVE ( 'NONE', #8251, #9836, #21584, .T. ) ;
#18431=EDGE_LOOP ( 'NONE', ( #13207, #20233 ) ) ;
#18535=EDGE_LOOP ( 'NONE', ( #16265, #5486, #14803, #19791 ) ) ;
#18600=CYLINDRICAL_SURFACE ( 'NONE', #21690, 10.49999999999999822 ) ;
#18684=FILL_AREA_STYLE ('',( #5737 ) ) ;
#18719=ADVANCED_FACE ( 'NONE', ( #8966, #6005 ), #3999, .T. ) ;
#18837=DIRECTION ( 'NONE',  ( -0.000000000000000000, -0.000000000000000000, -1.000000000000000000 ) ) ;
#18845=CIRCLE ( 'NONE', #12131, 10.49999999999999822 ) ;
#19024=VERTEX_POINT ( 'NONE', #17438 ) ;
#19048=ORIENTED_EDGE ( 'NONE', *, *, #12699, .F. ) ;
#19076=CARTESIAN_POINT ( 'NONE',  ( 0.000000000000000000, 0.000000000000000000, 0.000000000000000000 ) ) ;
#19172=EDGE_CURVE ( 'NONE', #4094, #19024, #330, .T. ) ;
#19241=CARTESIAN_POINT ( 'NONE',  ( 0.000000000000000000, 0.000000000000000000, 3.000000000000000000 ) ) ;
#19248=CARTESIAN_POINT ( 'NONE',  ( -6.500000000000014211, 60.00000000000001421, 0.000000000000000000 ) ) ;
#19257=VECTOR ( 'NONE', #16856, 1000.000000000000000 ) ;
#19377=CYLINDRICAL_SURFACE ( 'NONE', #10155, 120.0000000000000000 ) ;
#19390=CARTESIAN_POINT ( 'NONE',  ( -7.500000000000000000, 0.000000000000000000, 0.000000000000000000 ) ) ;
#19417=ORIENTED_EDGE ( 'NONE', *, *, #18346, .F. ) ;
#19579=ORIENTED_EDGE ( 'NONE', *, *, #1097, .T. ) ;
#19593=DIRECTION ( 'NONE',  ( 0.000000000000000000, 0.000000000000000000, -1.000000000000000000 ) ) ;
#19618=ORIENTED_EDGE ( 'NONE', *, *, #8911, .F. ) ;
#19619=EDGE_CURVE ( 'NONE', #2060, #2977, #19820, .T. ) ;
#19678=PRODUCT_DEFINITION ( 'UNKNOWN', '', #17697, #8727 ) ;
#19718=DIRECTION ( 'NONE',  ( -0.000000000000000000, -0.000000000000000000, -1.000000000000000000 ) ) ;
#19791=ORIENTED_EDGE ( 'NONE', *, *, #11613, .T. ) ;
#19820=LINE ( 'NONE', #13180, #4936 ) ;
#19915=AXIS2_PLACEMENT_3D ( 'NONE', #2468, #3797, #9193 ) ;
#19917=DIRECTION ( 'NONE',  ( 0.000000000000000000, 0.000000000000000000, -1.000000000000000000 ) ) ;
#19920=CARTESIAN_POINT ( 'NONE',  ( 0.000000000000000000, 0.000000000000000000, 3.000000000000000000 ) ) ;
#19939=ORIENTED_EDGE ( 'NONE', *, *, #20276, .F. ) ;
#19951=ADVANCED_FACE ( 'NONE', ( #587 ), #16154, .T. ) ;
#20023=ORIENTED_EDGE ( 'NONE', *, *, #20276, .T. ) ;
#20106=CARTESIAN_POINT ( 'NONE',  ( 123.0000000000000000, 0.000000000000000000, -3.000000000000000000 ) ) ;
#20137=EDGE_LOOP ( 'NONE', ( #19048, #7834, #10063, #11629 ) ) ;
#20147=DIRECTION ( 'NONE',  ( -1.000000000000000000, 0.000000000000000000, 0.000000000000000000 ) ) ;
#20187=DIRECTION ( 'NONE',  ( 0.000000000000000000, 0.000000000000000000, 1.000000000000000000 ) ) ;
#20211=VERTEX_POINT ( 'NONE', #13483 ) ;
#20227=( GEOMETRIC_REPRESENTATION_CONTEXT ( 3 ) GLOBAL_UNCERTAINTY_ASSIGNED_CONTEXT ( ( #3051 ) ) GLOBAL_UNIT_ASSIGNED_CONTEXT ( ( #12039, #10369, #4401 ) ) REPRESENTATION_CONTEXT ( 'NONE', 'WORKASPACE' ) );
#20233=ORIENTED_EDGE ( 'NONE', *, *, #10919, .F. ) ;
#20238=AXIS2_PLACEMENT_3D ( 'NONE', #11640, #16705, #7882 ) ;
#20273=CARTESIAN_POINT ( 'NONE',  ( 0.000000000000000000, 0.000000000000000000, -3.000000000000000000 ) ) ;
#20276=EDGE_CURVE ( 'NONE', #3553, #4094, #12027, .T. ) ;
#20295=CIRCLE ( 'NONE', #5468, 7.500000000000000000 ) ;
#20579=EDGE_LOOP ( 'NONE', ( #20690, #16590 ) ) ;
#20607=CIRCLE ( 'NONE', #17078, 120.0000000000000000 ) ;
#20616=VERTEX_POINT ( 'NONE', #9345 ) ;
#20690=ORIENTED_EDGE ( 'NONE', *, *, #13236, .T. ) ;
#20844=DIRECTION ( 'NONE',  ( -1.000000000000000000, 0.000000000000000000, 0.000000000000000000 ) ) ;
#20851=DIRECTION ( 'NONE',  ( -0.000000000000000000, -0.000000000000000000, -1.000000000000000000 ) ) ;
#20872=CARTESIAN_POINT ( 'NONE',  ( 7.500000000000000000, 9.184850993605147944E-16, 0.000000000000000000 ) ) ;
#21017=DIRECTION ( 'NONE',  ( 1.000000000000000000, 0.000000000000000000, -0.000000000000000000 ) ) ;
#21171=ORIENTED_EDGE ( 'NONE', *, *, #2094, .T. ) ;
#21247=CARTESIAN_POINT ( 'NONE',  ( 0.000000000000000000, 0.000000000000000000, -3.000000000000000000 ) ) ;
#21397=AXIS2_PLACEMENT_3D ( 'NONE', #9409, #19593, #14282 ) ;
#21450=CIRCLE ( 'NONE', #15461, 120.0000000000000000 ) ;
#21507=CARTESIAN_POINT ( 'NONE',  ( -6.500000000000014211, 60.00000000000001421, -3.000000000000000000 ) ) ;
#21520=DIRECTION ( 'NONE',  ( 1.000000000000000000, 0.000000000000000000, 0.000000000000000000 ) ) ;
#21584=LINE ( 'NONE', #4797, #10845 ) ;
#21601=CARTESIAN_POINT ( 'NONE',  ( 120.0000000000000000, 0.000000000000000000, 25.00000000000000000 ) ) ;
#21614=DIRECTION ( 'NONE',  ( 0.000000000000000000, 0.000000000000000000, 1.000000000000000000 ) ) ;
#21615=ORIENTED_EDGE ( 'NONE', *, *, #15442, .F. ) ;
#21642=ADVANCED_FACE ( 'NONE', ( #9789 ), #17993, .F. ) ;
#21674=CIRCLE ( 'NONE', #14970, 7.500000000000000000 ) ;
#21681=FACE_BOUND ( 'NONE', #13358, .T. ) ;
#21683=CARTESIAN_POINT ( 'NONE',  ( 0.000000000000000000, 0.000000000000000000, 0.000000000000000000 ) ) ;
#21690=AXIS2_PLACEMENT_3D ( 'NONE', #10196, #1801, #17043 ) ;
#21702=CARTESIAN_POINT ( 'NONE',  ( -123.0000000000000000, 1.506315562951244531E-14, -3.000000000000000000 ) ) ;
#21837=CARTESIAN_POINT ( 'NONE',  ( 0.000000000000000000, 0.000000000000000000, 0.000000000000000000 ) ) ;
ENDSEC;
END-ISO-10303-21;
